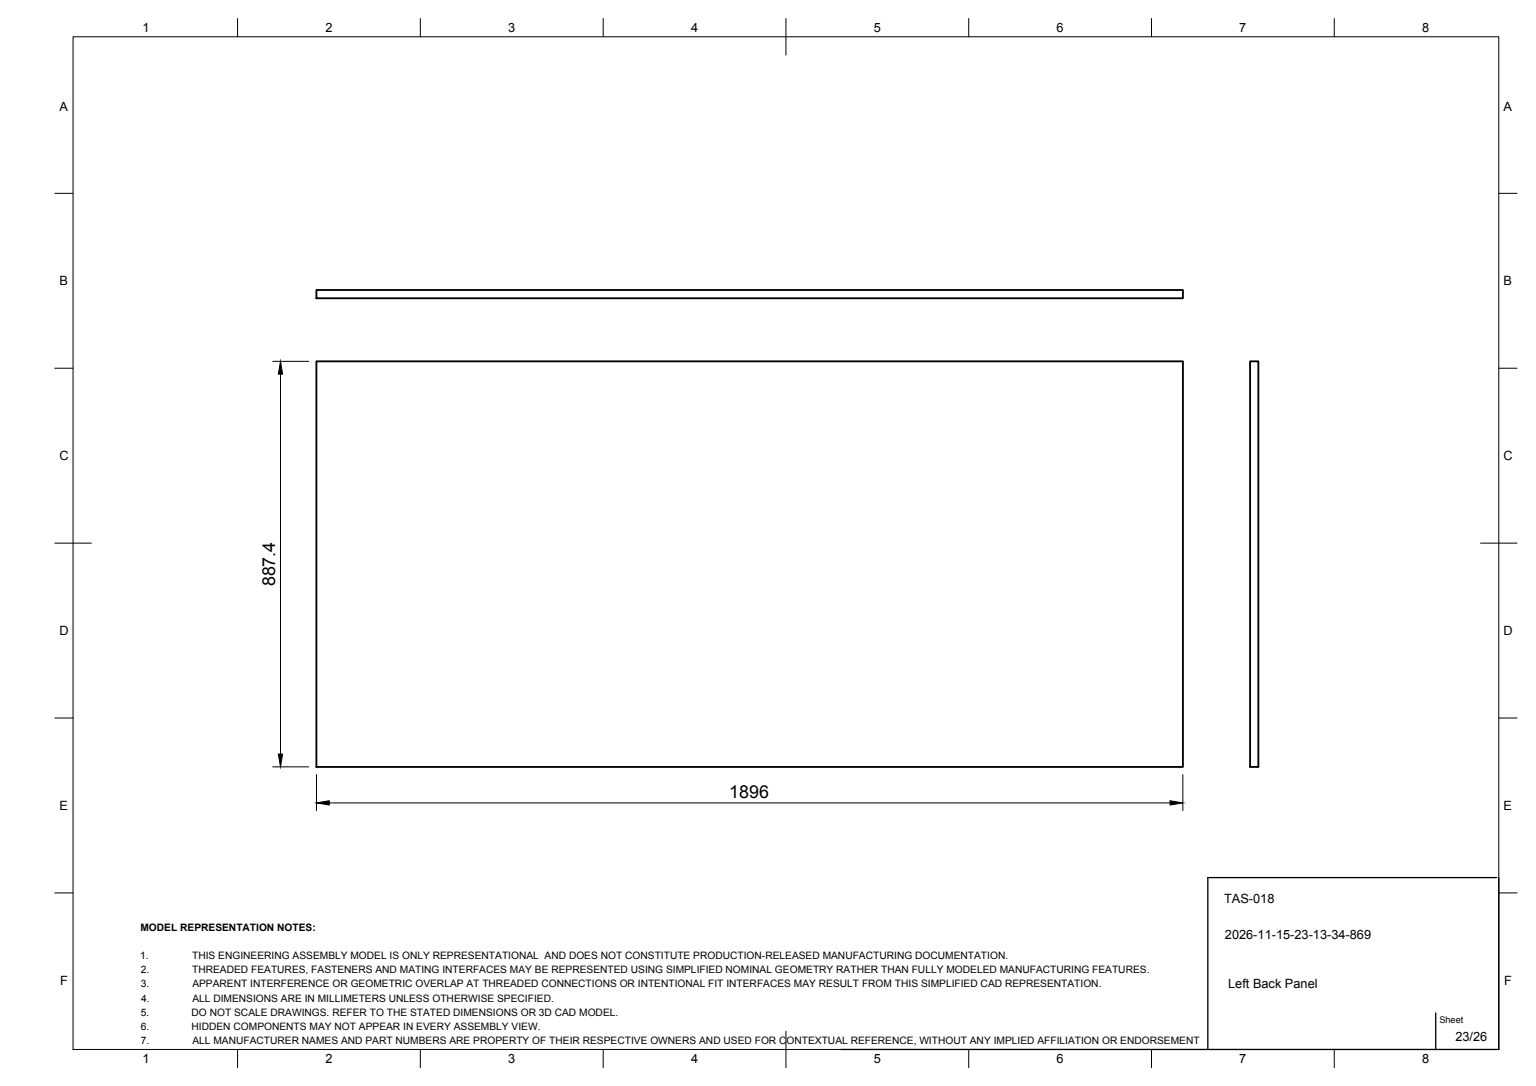
ISO-10303-21;
HEADER;
/* Generated by software containing ST-Developer
 * from STEP Tools, Inc. (www.steptools.com) 
 */

FILE_DESCRIPTION(
/* description */ (''),
/* implementation_level */ '2;1');

FILE_NAME(
/* name */ 'Left Back Panel.step',
/* time_stamp */ '2026-11-15T15:17:57-08:00',
/* author */ (''),
/* organization */ (''),
/* preprocessor_version */ 'ST-DEVELOPER v20.2',
/* originating_system */ 'Autodesk Translation Framework v15.17.0.0',
/* authorisation */ '');

FILE_SCHEMA (('AUTOMOTIVE_DESIGN { 1 0 10303 214 3 1 1 }'));
ENDSEC;

DATA;
#10=MECHANICAL_DESIGN_GEOMETRIC_PRESENTATION_REPRESENTATION('',(#198),#3723);
#150=SHAPE_REPRESENTATION_RELATIONSHIP('SRR','None',#3831,#174);
#174=ADVANCED_BREP_SHAPE_REPRESENTATION('',(#222),#3720);
#198=STYLED_ITEM('',(#3949),#222);
#222=MANIFOLD_SOLID_BREP('Body1',#2046);
#333=FACE_OUTER_BOUND('',#459,.T.);
#334=FACE_OUTER_BOUND('',#460,.T.);
#335=FACE_OUTER_BOUND('',#461,.T.);
#336=FACE_OUTER_BOUND('',#462,.T.);
#337=FACE_OUTER_BOUND('',#463,.T.);
#338=FACE_OUTER_BOUND('',#464,.T.);
#459=EDGE_LOOP('',(#1707,#1708,#1709,#1710));
#460=EDGE_LOOP('',(#1711,#1712,#1713,#1714));
#461=EDGE_LOOP('',(#1715,#1716,#1717,#1718));
#462=EDGE_LOOP('',(#1719,#1720,#1721,#1722));
#463=EDGE_LOOP('',(#1723,#1724,#1725,#1726));
#464=EDGE_LOOP('',(#1727,#1728,#1729,#1730));
#663=LINE('',#3569,#885);
#664=LINE('',#3571,#886);
#665=LINE('',#3573,#887);
#666=LINE('',#3574,#888);
#667=LINE('',#3577,#889);
#668=LINE('',#3579,#890);
#669=LINE('',#3580,#891);
#670=LINE('',#3583,#892);
#671=LINE('',#3585,#893);
#672=LINE('',#3586,#894);
#673=LINE('',#3588,#895);
#674=LINE('',#3589,#896);
#885=VECTOR('',#2981,74.6456692913386);
#886=VECTOR('',#2982,0.708661417322834);
#887=VECTOR('',#2983,74.6456692913386);
#888=VECTOR('',#2984,0.708661417322834);
#889=VECTOR('',#2987,34.9370078740157);
#890=VECTOR('',#2988,0.708661417322834);
#891=VECTOR('',#2989,34.9370078740157);
#892=VECTOR('',#2992,74.6456692913386);
#893=VECTOR('',#2993,0.708661417322834);
#894=VECTOR('',#2994,74.6456692913386);
#895=VECTOR('',#2997,34.9370078740157);
#896=VECTOR('',#2998,34.9370078740157);
#1053=VERTEX_POINT('',#3567);
#1054=VERTEX_POINT('',#3568);
#1055=VERTEX_POINT('',#3570);
#1056=VERTEX_POINT('',#3572);
#1057=VERTEX_POINT('',#3576);
#1058=VERTEX_POINT('',#3578);
#1059=VERTEX_POINT('',#3582);
#1060=VERTEX_POINT('',#3584);
#1275=EDGE_CURVE('',#1053,#1054,#663,.T.);
#1276=EDGE_CURVE('',#1055,#1054,#664,.T.);
#1277=EDGE_CURVE('',#1056,#1055,#665,.T.);
#1278=EDGE_CURVE('',#1056,#1053,#666,.T.);
#1279=EDGE_CURVE('',#1054,#1057,#667,.T.);
#1280=EDGE_CURVE('',#1058,#1057,#668,.T.);
#1281=EDGE_CURVE('',#1055,#1058,#669,.T.);
#1282=EDGE_CURVE('',#1057,#1059,#670,.T.);
#1283=EDGE_CURVE('',#1060,#1059,#671,.T.);
#1284=EDGE_CURVE('',#1058,#1060,#672,.T.);
#1285=EDGE_CURVE('',#1059,#1053,#673,.T.);
#1286=EDGE_CURVE('',#1060,#1056,#674,.T.);
#1707=ORIENTED_EDGE('',*,*,#1275,.T.);
#1708=ORIENTED_EDGE('',*,*,#1276,.F.);
#1709=ORIENTED_EDGE('',*,*,#1277,.F.);
#1710=ORIENTED_EDGE('',*,*,#1278,.T.);
#1711=ORIENTED_EDGE('',*,*,#1279,.T.);
#1712=ORIENTED_EDGE('',*,*,#1280,.F.);
#1713=ORIENTED_EDGE('',*,*,#1281,.F.);
#1714=ORIENTED_EDGE('',*,*,#1276,.T.);
#1715=ORIENTED_EDGE('',*,*,#1282,.T.);
#1716=ORIENTED_EDGE('',*,*,#1283,.F.);
#1717=ORIENTED_EDGE('',*,*,#1284,.F.);
#1718=ORIENTED_EDGE('',*,*,#1280,.T.);
#1719=ORIENTED_EDGE('',*,*,#1285,.T.);
#1720=ORIENTED_EDGE('',*,*,#1278,.F.);
#1721=ORIENTED_EDGE('',*,*,#1286,.F.);
#1722=ORIENTED_EDGE('',*,*,#1283,.T.);
#1723=ORIENTED_EDGE('',*,*,#1277,.T.);
#1724=ORIENTED_EDGE('',*,*,#1281,.T.);
#1725=ORIENTED_EDGE('',*,*,#1284,.T.);
#1726=ORIENTED_EDGE('',*,*,#1286,.T.);
#1727=ORIENTED_EDGE('',*,*,#1275,.F.);
#1728=ORIENTED_EDGE('',*,*,#1285,.F.);
#1729=ORIENTED_EDGE('',*,*,#1282,.F.);
#1730=ORIENTED_EDGE('',*,*,#1279,.F.);
#1881=PLANE('',#2459);
#1882=PLANE('',#2460);
#1883=PLANE('',#2461);
#1884=PLANE('',#2462);
#1885=PLANE('',#2463);
#1886=PLANE('',#2464);
#2007=ADVANCED_FACE('',(#333),#1881,.F.);
#2008=ADVANCED_FACE('',(#334),#1882,.F.);
#2009=ADVANCED_FACE('',(#335),#1883,.F.);
#2010=ADVANCED_FACE('',(#336),#1884,.F.);
#2011=ADVANCED_FACE('',(#337),#1885,.T.);
#2012=ADVANCED_FACE('',(#338),#1886,.F.);
#2046=CLOSED_SHELL('',(#2007,#2008,#2009,#2010,#2011,#2012));
#2458=AXIS2_PLACEMENT_3D('',#3565,#2977,#2978);
#2459=AXIS2_PLACEMENT_3D('',#3566,#2979,#2980);
#2460=AXIS2_PLACEMENT_3D('',#3575,#2985,#2986);
#2461=AXIS2_PLACEMENT_3D('',#3581,#2990,#2991);
#2462=AXIS2_PLACEMENT_3D('',#3587,#2995,#2996);
#2463=AXIS2_PLACEMENT_3D('',#3590,#2999,#3000);
#2464=AXIS2_PLACEMENT_3D('',#3591,#3001,#3002);
#2977=DIRECTION('axis',(0.,0.,1.));
#2978=DIRECTION('refdir',(1.,0.,0.));
#2979=DIRECTION('center_axis',(1.,1.17112133399278E-16,0.));
#2980=DIRECTION('ref_axis',(0.,0.,-1.));
#2981=DIRECTION('',(1.49903530751076E-16,-1.,0.));
#2982=DIRECTION('',(0.,0.,-1.));
#2983=DIRECTION('',(1.49903530751076E-16,-1.,0.));
#2984=DIRECTION('',(0.,0.,-1.));
#2985=DIRECTION('center_axis',(0.,1.,0.));
#2986=DIRECTION('ref_axis',(0.,0.,1.));
#2987=DIRECTION('',(1.,0.,0.));
#2988=DIRECTION('',(0.,0.,-1.));
#2989=DIRECTION('',(1.,0.,0.));
#2990=DIRECTION('center_axis',(-1.,-9.88133625556409E-17,0.));
#2991=DIRECTION('ref_axis',(0.,0.,1.));
#2992=DIRECTION('',(-9.895975272239E-17,1.,0.));
#2993=DIRECTION('',(0.,0.,-1.));
#2994=DIRECTION('',(-9.895975272239E-17,1.,0.));
#2995=DIRECTION('center_axis',(0.,-1.,0.));
#2996=DIRECTION('ref_axis',(0.,0.,-1.));
#2997=DIRECTION('',(-1.,0.,0.));
#2998=DIRECTION('',(-1.,0.,0.));
#2999=DIRECTION('center_axis',(0.,0.,1.));
#3000=DIRECTION('ref_axis',(1.,0.,0.));
#3001=DIRECTION('center_axis',(0.,0.,1.));
#3002=DIRECTION('ref_axis',(1.,0.,0.));
#3565=CARTESIAN_POINT('',(0.,0.,0.));
#3566=CARTESIAN_POINT('Origin',(-35.2913385826772,79.2913385826772,0.708661417322834));
#3567=CARTESIAN_POINT('',(-35.2913385826772,79.2913385826772,0.));
#3568=CARTESIAN_POINT('',(-35.2913385826772,4.64566929133858,0.));
#3569=CARTESIAN_POINT('',(-35.2913385826772,79.2913385826772,0.));
#3570=CARTESIAN_POINT('',(-35.2913385826772,4.64566929133858,0.708661417322834));
#3571=CARTESIAN_POINT('',(-35.2913385826772,4.64566929133858,0.708661417322834));
#3572=CARTESIAN_POINT('',(-35.2913385826772,79.2913385826772,0.708661417322834));
#3573=CARTESIAN_POINT('',(-35.2913385826772,79.2913385826772,0.708661417322834));
#3574=CARTESIAN_POINT('',(-35.2913385826772,79.2913385826772,0.708661417322834));
#3575=CARTESIAN_POINT('Origin',(-35.2913385826772,4.64566929133858,0.708661417322834));
#3576=CARTESIAN_POINT('',(-0.354330708661419,4.64566929133858,0.));
#3577=CARTESIAN_POINT('',(-35.2913385826772,4.64566929133858,0.));
#3578=CARTESIAN_POINT('',(-0.354330708661419,4.64566929133858,0.708661417322834));
#3579=CARTESIAN_POINT('',(-0.354330708661419,4.64566929133858,0.708661417322834));
#3580=CARTESIAN_POINT('',(-35.2913385826772,4.64566929133858,0.708661417322834));
#3581=CARTESIAN_POINT('Origin',(-0.354330708661426,79.2913385826772,0.708661417322834));
#3582=CARTESIAN_POINT('',(-0.354330708661426,79.2913385826772,0.));
#3583=CARTESIAN_POINT('',(-0.354330708661419,4.64566929133858,0.));
#3584=CARTESIAN_POINT('',(-0.354330708661426,79.2913385826772,0.708661417322834));
#3585=CARTESIAN_POINT('',(-0.354330708661426,79.2913385826772,0.708661417322834));
#3586=CARTESIAN_POINT('',(-0.354330708661419,4.64566929133858,0.708661417322834));
#3587=CARTESIAN_POINT('Origin',(-35.2913385826772,79.2913385826772,0.708661417322834));
#3588=CARTESIAN_POINT('',(-0.354330708661426,79.2913385826772,0.));
#3589=CARTESIAN_POINT('',(-0.354330708661426,79.2913385826772,0.708661417322834));
#3590=CARTESIAN_POINT('Origin',(0.,0.,0.708661417322834));
#3591=CARTESIAN_POINT('Origin',(0.,0.,0.));
#3693=UNCERTAINTY_MEASURE_WITH_UNIT(LENGTH_MEASURE(0.000393700787401575),
#3725,'DISTANCE_ACCURACY_VALUE',
'Maximum model space distance between geometric entities at asserted c
onnectivities');
#3696=UNCERTAINTY_MEASURE_WITH_UNIT(LENGTH_MEASURE(0.000393700787401575),
#3725,'DISTANCE_ACCURACY_VALUE',
'Maximum model space distance between geometric entities at asserted c
onnectivities');
#3720=(
GEOMETRIC_REPRESENTATION_CONTEXT(3)
GLOBAL_UNCERTAINTY_ASSIGNED_CONTEXT((#3693))
GLOBAL_UNIT_ASSIGNED_CONTEXT((#3725,#3729,#3730))
REPRESENTATION_CONTEXT('','3D')
);
#3723=(
GEOMETRIC_REPRESENTATION_CONTEXT(3)
GLOBAL_UNCERTAINTY_ASSIGNED_CONTEXT((#3696))
GLOBAL_UNIT_ASSIGNED_CONTEXT((#3725,#3729,#3730))
REPRESENTATION_CONTEXT('','3D')
);
#3724=DIMENSIONAL_EXPONENTS(1.,0.,0.,0.,0.,0.,0.);
#3725=(
CONVERSION_BASED_UNIT('inch',#3728)
LENGTH_UNIT()
NAMED_UNIT(#3724)
);
#3726=(
LENGTH_UNIT()
NAMED_UNIT(*)
SI_UNIT(.MILLI.,.METRE.)
);
#3728=LENGTH_MEASURE_WITH_UNIT(LENGTH_MEASURE(25.4),#3726);
#3729=(
NAMED_UNIT(*)
PLANE_ANGLE_UNIT()
SI_UNIT($,.RADIAN.)
);
#3730=(
NAMED_UNIT(*)
SI_UNIT($,.STERADIAN.)
SOLID_ANGLE_UNIT()
);
#3754=SHAPE_DEFINITION_REPRESENTATION(#3781,#3831);
#3781=PRODUCT_DEFINITION_SHAPE('',$,#3858);
#3831=SHAPE_REPRESENTATION('',(#2458),#3720);
#3834=PRODUCT_DEFINITION_CONTEXT('part definition',#3914,'design');
#3858=PRODUCT_DEFINITION('2026-11-15-23-13-34-869','Left Back Panel',#3884,
#3834);
#3884=PRODUCT_DEFINITION_FORMATION('',$,#3939);
#3914=APPLICATION_CONTEXT(
'Core Data for Automotive Mechanical Design Process');
#3915=PRODUCT_CONTEXT('part definition',#3914,'mechanical');
#3939=PRODUCT('2026-11-15-23-13-34-869','Left Back Panel',$,(#3915));
#3949=PRESENTATION_STYLE_ASSIGNMENT((#3957));
#3957=SURFACE_STYLE_USAGE(.BOTH.,#3965);
#3965=SURFACE_SIDE_STYLE('',(#3973));
#3973=SURFACE_STYLE_FILL_AREA(#3981);
#3981=FILL_AREA_STYLE('Sky Blue',(#3989));
#3989=FILL_AREA_STYLE_COLOUR('Sky Blue',#3997);
#3997=COLOUR_RGB('Sky Blue',0.529411764705882,0.807843137254902,0.92156862745098);
ENDSEC;
END-ISO-10303-21;
